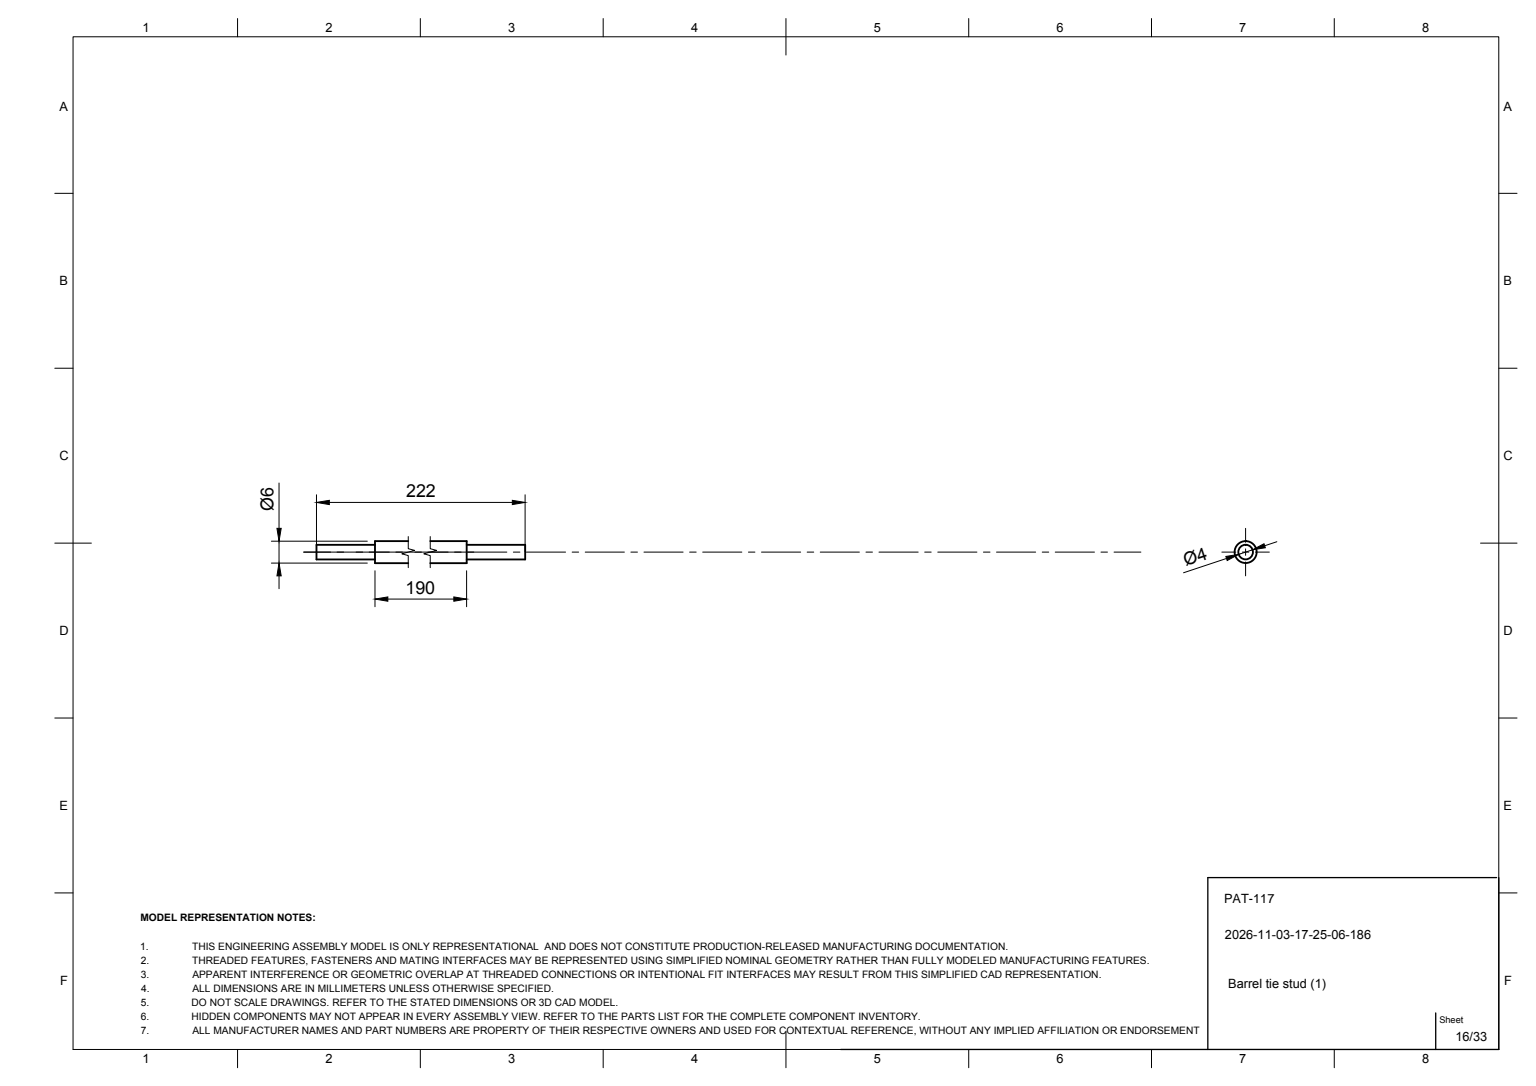
ISO-10303-21;
HEADER;
/* Generated by software containing ST-Developer
 * from STEP Tools, Inc. (www.steptools.com) 
 */

FILE_DESCRIPTION(
/* description */ ('Counterbalanced vertical column'),
/* implementation_level */ '2;1');

FILE_NAME(
/* name */ 'Barrel tie stud (1).step',
/* time_stamp */ '2026-10-29T16:47:22-07:00',
/* author */ (''),
/* organization */ (''),
/* preprocessor_version */ 'ST-DEVELOPER v20.2',
/* originating_system */ 'Autodesk Translation Framework v15.17.0.0',
/* authorisation */ '');

FILE_SCHEMA (('AUTOMOTIVE_DESIGN { 1 0 10303 214 3 1 1 }'));
ENDSEC;

DATA;
#10=MECHANICAL_DESIGN_GEOMETRIC_PRESENTATION_REPRESENTATION('',(#362),#15040);
#292=SHAPE_REPRESENTATION_RELATIONSHIP('SRR','None',#15196,#327);
#327=ADVANCED_BREP_SHAPE_REPRESENTATION('',(#397),#15015);
#362=STYLED_ITEM('',(#15464),#397);
#397=MANIFOLD_SOLID_BREP('Body1',#7085);
#464=FACE_BOUND('',#1380,.T.);
#465=FACE_BOUND('',#1382,.T.);
#597=PLANE('',#7681);
#598=PLANE('',#7684);
#599=PLANE('',#7692);
#600=PLANE('',#7693);
#926=FACE_OUTER_BOUND('',#1379,.T.);
#927=FACE_OUTER_BOUND('',#1381,.T.);
#928=FACE_OUTER_BOUND('',#1383,.T.);
#929=FACE_OUTER_BOUND('',#1384,.T.);
#930=FACE_OUTER_BOUND('',#1385,.T.);
#931=FACE_OUTER_BOUND('',#1386,.T.);
#932=FACE_OUTER_BOUND('',#1387,.T.);
#1379=EDGE_LOOP('',(#5184));
#1380=EDGE_LOOP('',(#5185));
#1381=EDGE_LOOP('',(#5186));
#1382=EDGE_LOOP('',(#5187));
#1383=EDGE_LOOP('',(#5188,#5189,#5190,#5191));
#1384=EDGE_LOOP('',(#5192,#5193,#5194,#5195));
#1385=EDGE_LOOP('',(#5196,#5197,#5198,#5199));
#1386=EDGE_LOOP('',(#5200));
#1387=EDGE_LOOP('',(#5201));
#1881=LINE('',#10794,#2552);
#1882=LINE('',#10797,#2553);
#1883=LINE('',#10802,#2554);
#2552=VECTOR('',#8731,0.3);
#2553=VECTOR('',#8734,0.2);
#2554=VECTOR('',#8741,0.2);
#3161=CIRCLE('',#7682,0.3);
#3162=CIRCLE('',#7683,0.2);
#3163=CIRCLE('',#7685,0.3);
#3164=CIRCLE('',#7686,0.2);
#3165=CIRCLE('',#7689,0.2);
#3166=CIRCLE('',#7691,0.2);
#3438=VERTEX_POINT('',#10784);
#3439=VERTEX_POINT('',#10786);
#3440=VERTEX_POINT('',#10789);
#3441=VERTEX_POINT('',#10791);
#3442=VERTEX_POINT('',#10796);
#3443=VERTEX_POINT('',#10800);
#4093=EDGE_CURVE('',#3438,#3438,#3161,.T.);
#4094=EDGE_CURVE('',#3439,#3439,#3162,.T.);
#4095=EDGE_CURVE('',#3440,#3440,#3163,.T.);
#4096=EDGE_CURVE('',#3441,#3441,#3164,.T.);
#4097=EDGE_CURVE('',#3438,#3440,#1881,.T.);
#4098=EDGE_CURVE('',#3441,#3442,#1882,.T.);
#4099=EDGE_CURVE('',#3442,#3442,#3165,.T.);
#4100=EDGE_CURVE('',#3443,#3443,#3166,.T.);
#4101=EDGE_CURVE('',#3443,#3439,#1883,.T.);
#5184=ORIENTED_EDGE('',*,*,#4093,.T.);
#5185=ORIENTED_EDGE('',*,*,#4094,.F.);
#5186=ORIENTED_EDGE('',*,*,#4095,.F.);
#5187=ORIENTED_EDGE('',*,*,#4096,.F.);
#5188=ORIENTED_EDGE('',*,*,#4093,.F.);
#5189=ORIENTED_EDGE('',*,*,#4097,.T.);
#5190=ORIENTED_EDGE('',*,*,#4095,.T.);
#5191=ORIENTED_EDGE('',*,*,#4097,.F.);
#5192=ORIENTED_EDGE('',*,*,#4096,.T.);
#5193=ORIENTED_EDGE('',*,*,#4098,.T.);
#5194=ORIENTED_EDGE('',*,*,#4099,.T.);
#5195=ORIENTED_EDGE('',*,*,#4098,.F.);
#5196=ORIENTED_EDGE('',*,*,#4100,.F.);
#5197=ORIENTED_EDGE('',*,*,#4101,.T.);
#5198=ORIENTED_EDGE('',*,*,#4094,.T.);
#5199=ORIENTED_EDGE('',*,*,#4101,.F.);
#5200=ORIENTED_EDGE('',*,*,#4100,.T.);
#5201=ORIENTED_EDGE('',*,*,#4099,.F.);
#6608=CYLINDRICAL_SURFACE('',#7687,0.3);
#6609=CYLINDRICAL_SURFACE('',#7688,0.2);
#6610=CYLINDRICAL_SURFACE('',#7690,0.2);
#6768=ADVANCED_FACE('',(#926,#464),#597,.T.);
#6769=ADVANCED_FACE('',(#927,#465),#598,.F.);
#6770=ADVANCED_FACE('',(#928),#6608,.T.);
#6771=ADVANCED_FACE('',(#929),#6609,.T.);
#6772=ADVANCED_FACE('',(#930),#6610,.T.);
#6773=ADVANCED_FACE('',(#931),#599,.T.);
#6774=ADVANCED_FACE('',(#932),#600,.F.);
#7085=CLOSED_SHELL('',(#6768,#6769,#6770,#6771,#6772,#6773,#6774));
#7680=AXIS2_PLACEMENT_3D('',#10782,#8715,#8716);
#7681=AXIS2_PLACEMENT_3D('',#10783,#8717,#8718);
#7682=AXIS2_PLACEMENT_3D('',#10785,#8719,#8720);
#7683=AXIS2_PLACEMENT_3D('',#10787,#8721,#8722);
#7684=AXIS2_PLACEMENT_3D('',#10788,#8723,#8724);
#7685=AXIS2_PLACEMENT_3D('',#10790,#8725,#8726);
#7686=AXIS2_PLACEMENT_3D('',#10792,#8727,#8728);
#7687=AXIS2_PLACEMENT_3D('',#10793,#8729,#8730);
#7688=AXIS2_PLACEMENT_3D('',#10795,#8732,#8733);
#7689=AXIS2_PLACEMENT_3D('',#10798,#8735,#8736);
#7690=AXIS2_PLACEMENT_3D('',#10799,#8737,#8738);
#7691=AXIS2_PLACEMENT_3D('',#10801,#8739,#8740);
#7692=AXIS2_PLACEMENT_3D('',#10803,#8742,#8743);
#7693=AXIS2_PLACEMENT_3D('',#10804,#8744,#8745);
#8715=DIRECTION('axis',(0.,0.,1.));
#8716=DIRECTION('refdir',(1.,0.,0.));
#8717=DIRECTION('center_axis',(0.,0.,1.));
#8718=DIRECTION('ref_axis',(1.,0.,0.));
#8719=DIRECTION('center_axis',(0.,0.,1.));
#8720=DIRECTION('ref_axis',(1.,0.,0.));
#8721=DIRECTION('center_axis',(0.,0.,1.));
#8722=DIRECTION('ref_axis',(1.,0.,0.));
#8723=DIRECTION('center_axis',(0.,0.,1.));
#8724=DIRECTION('ref_axis',(1.,0.,0.));
#8725=DIRECTION('center_axis',(0.,0.,1.));
#8726=DIRECTION('ref_axis',(1.,0.,0.));
#8727=DIRECTION('center_axis',(0.,0.,-1.));
#8728=DIRECTION('ref_axis',(1.,0.,0.));
#8729=DIRECTION('center_axis',(0.,0.,1.));
#8730=DIRECTION('ref_axis',(1.,0.,0.));
#8731=DIRECTION('',(0.,0.,-1.));
#8732=DIRECTION('center_axis',(0.,0.,1.));
#8733=DIRECTION('ref_axis',(1.,0.,0.));
#8734=DIRECTION('',(0.,0.,-1.));
#8735=DIRECTION('center_axis',(0.,0.,1.));
#8736=DIRECTION('ref_axis',(1.,0.,0.));
#8737=DIRECTION('center_axis',(0.,0.,1.));
#8738=DIRECTION('ref_axis',(1.,0.,0.));
#8739=DIRECTION('center_axis',(0.,0.,1.));
#8740=DIRECTION('ref_axis',(1.,0.,0.));
#8741=DIRECTION('',(0.,0.,-1.));
#8742=DIRECTION('center_axis',(0.,0.,1.));
#8743=DIRECTION('ref_axis',(1.,0.,0.));
#8744=DIRECTION('center_axis',(0.,0.,1.));
#8745=DIRECTION('ref_axis',(1.,0.,0.));
#10782=CARTESIAN_POINT('',(0.,0.,0.));
#10783=CARTESIAN_POINT('Origin',(-5.2,0.,20.));
#10784=CARTESIAN_POINT('',(-5.5,-3.67394039744206E-17,20.));
#10785=CARTESIAN_POINT('Origin',(-5.2,0.,20.));
#10786=CARTESIAN_POINT('',(-5.4,-2.44929359829471E-17,20.));
#10787=CARTESIAN_POINT('Origin',(-5.2,0.,20.));
#10788=CARTESIAN_POINT('Origin',(-5.2,0.,1.));
#10789=CARTESIAN_POINT('',(-5.5,-3.67394039744206E-17,1.));
#10790=CARTESIAN_POINT('Origin',(-5.2,0.,1.));
#10791=CARTESIAN_POINT('',(-5.4,2.44929359829471E-17,1.));
#10792=CARTESIAN_POINT('Origin',(-5.2,0.,1.));
#10793=CARTESIAN_POINT('Origin',(-5.2,0.,1.));
#10794=CARTESIAN_POINT('',(-5.5,-3.67394039744206E-17,1.));
#10795=CARTESIAN_POINT('Origin',(-5.2,0.,-0.6));
#10796=CARTESIAN_POINT('',(-5.4,-2.44929359829471E-17,-0.6));
#10797=CARTESIAN_POINT('',(-5.4,-2.44929359829471E-17,-0.6));
#10798=CARTESIAN_POINT('Origin',(-5.2,0.,-0.6));
#10799=CARTESIAN_POINT('Origin',(-5.2,0.,-0.6));
#10800=CARTESIAN_POINT('',(-5.4,-2.44929359829471E-17,21.6));
#10801=CARTESIAN_POINT('Origin',(-5.2,0.,21.6));
#10802=CARTESIAN_POINT('',(-5.4,-2.44929359829471E-17,-0.6));
#10803=CARTESIAN_POINT('Origin',(-5.2,0.,21.6));
#10804=CARTESIAN_POINT('Origin',(-5.2,0.,-0.6));
#14975=UNCERTAINTY_MEASURE_WITH_UNIT(LENGTH_MEASURE(0.001),#15041,
'DISTANCE_ACCURACY_VALUE',
'Maximum model space distance between geometric entities at asserted c
onnectivities');
#15000=UNCERTAINTY_MEASURE_WITH_UNIT(LENGTH_MEASURE(0.001),#15041,
'DISTANCE_ACCURACY_VALUE',
'Maximum model space distance between geometric entities at asserted c
onnectivities');
#15015=(
GEOMETRIC_REPRESENTATION_CONTEXT(3)
GLOBAL_UNCERTAINTY_ASSIGNED_CONTEXT((#14975))
GLOBAL_UNIT_ASSIGNED_CONTEXT((#15041,#15043,#15044))
REPRESENTATION_CONTEXT('','3D')
);
#15040=(
GEOMETRIC_REPRESENTATION_CONTEXT(3)
GLOBAL_UNCERTAINTY_ASSIGNED_CONTEXT((#15000))
GLOBAL_UNIT_ASSIGNED_CONTEXT((#15041,#15043,#15044))
REPRESENTATION_CONTEXT('','3D')
);
#15041=(
LENGTH_UNIT()
NAMED_UNIT(*)
SI_UNIT(.CENTI.,.METRE.)
);
#15043=(
NAMED_UNIT(*)
PLANE_ANGLE_UNIT()
SI_UNIT($,.RADIAN.)
);
#15044=(
NAMED_UNIT(*)
SI_UNIT($,.STERADIAN.)
SOLID_ANGLE_UNIT()
);
#15059=SHAPE_DEFINITION_REPRESENTATION(#15098,#15196);
#15098=PRODUCT_DEFINITION_SHAPE('',$,#15236);
#15196=SHAPE_REPRESENTATION('',(#7680),#15015);
#15221=PRODUCT_DEFINITION_CONTEXT('part definition',#15340,'design');
#15236=PRODUCT_DEFINITION('Barrel tie stud (1)','Barrel tie stud (1)',#15275,
#15221);
#15275=PRODUCT_DEFINITION_FORMATION('',$,#15356);
#15340=APPLICATION_CONTEXT(
'Core Data for Automotive Mechanical Design Process');
#15341=PRODUCT_CONTEXT('part definition',#15340,'mechanical');
#15356=PRODUCT('Barrel tie stud (1)','Barrel tie stud (1)',
'Barrel tie stud (1)',(#15341));
#15458=COLOUR_RGB('Black',0.12,0.14,0.17);
#15459=FILL_AREA_STYLE_COLOUR('',#15458);
#15460=FILL_AREA_STYLE('',(#15459));
#15461=SURFACE_STYLE_FILL_AREA(#15460);
#15462=SURFACE_SIDE_STYLE('',(#15461));
#15463=SURFACE_STYLE_USAGE(.BOTH.,#15462);
#15464=PRESENTATION_STYLE_ASSIGNMENT((#15463));
ENDSEC;
END-ISO-10303-21;
